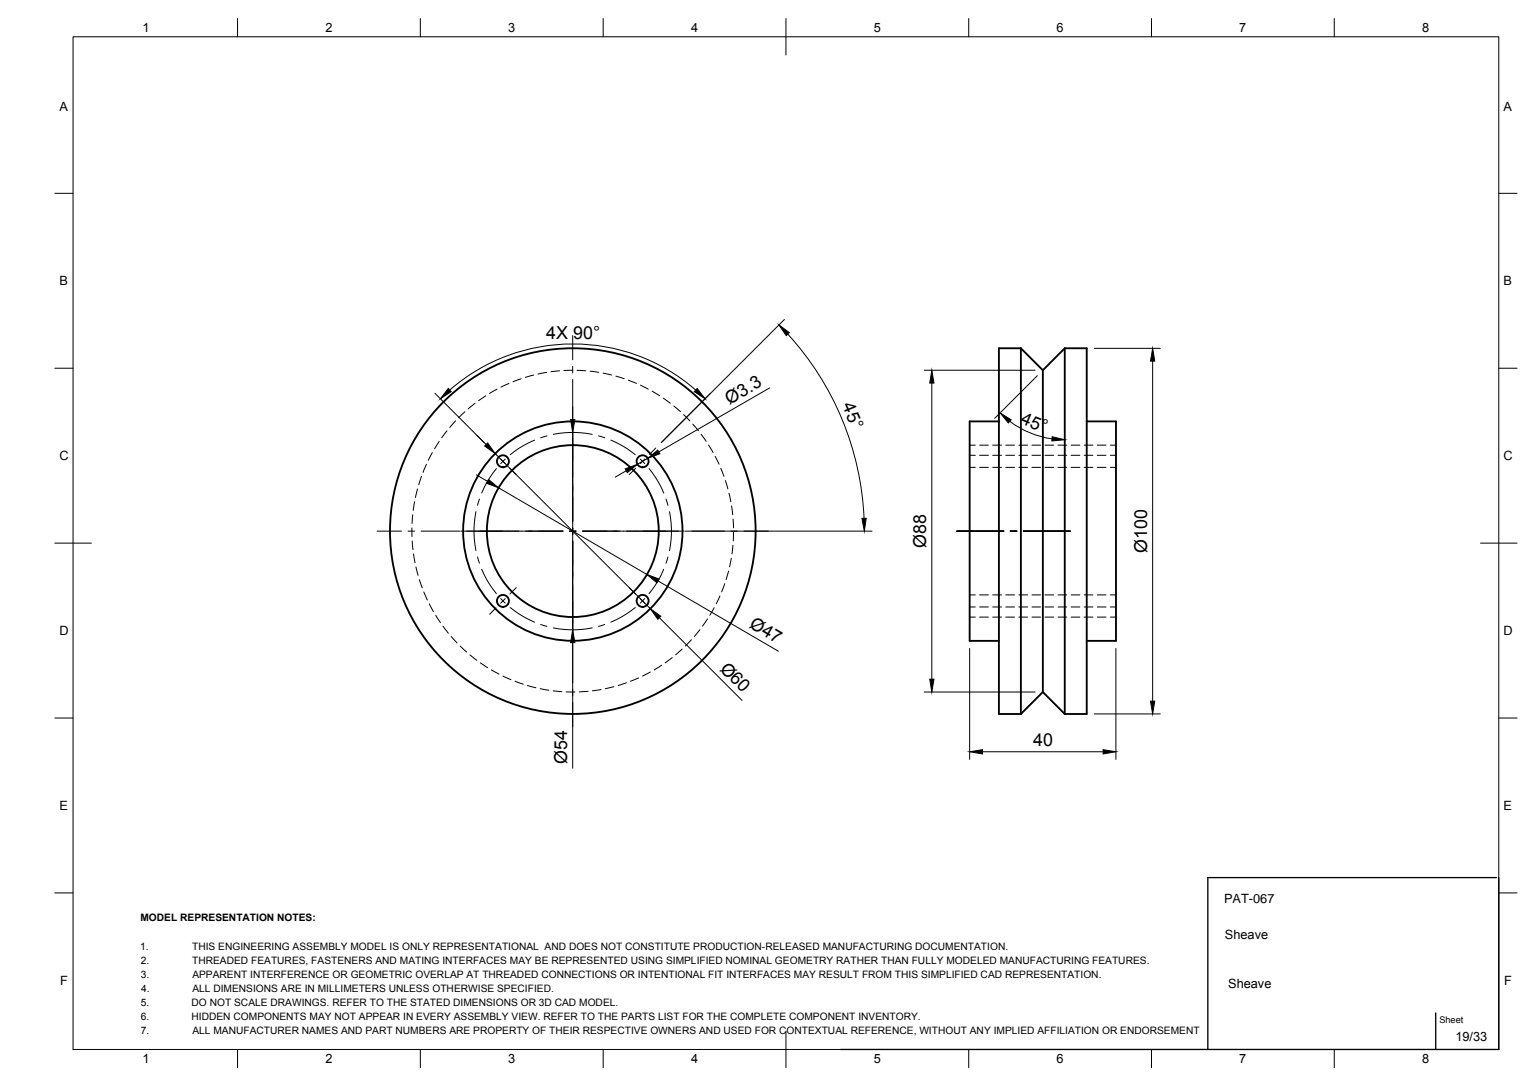
ISO-10303-21;
HEADER;
/* Generated by software containing ST-Developer
 * from STEP Tools, Inc. (www.steptools.com) 
 */

FILE_DESCRIPTION(
/* description */ ('Lifting hook block with sheave'),
/* implementation_level */ '2;1');

FILE_NAME(
/* name */ 'Sheave.step',
/* time_stamp */ '2026-10-28T03:23:54-07:00',
/* author */ (''),
/* organization */ (''),
/* preprocessor_version */ 'ST-DEVELOPER v20.2',
/* originating_system */ 'Autodesk Translation Framework v15.17.0.0',
/* authorisation */ '');

FILE_SCHEMA (('AUTOMOTIVE_DESIGN { 1 0 10303 214 3 1 1 }'));
ENDSEC;

DATA;
#10=MECHANICAL_DESIGN_GEOMETRIC_PRESENTATION_REPRESENTATION('',(#367),#9391);
#276=CONICAL_SURFACE('',#5601,4.7,0.785398163397448);
#277=CONICAL_SURFACE('',#5604,4.7,0.785398163397448);
#307=SHAPE_REPRESENTATION_RELATIONSHIP('SRR','None',#9539,#337);
#337=ADVANCED_BREP_SHAPE_REPRESENTATION('',(#403),#9374);
#367=STYLED_ITEM('',(#9752),#403);
#403=MANIFOLD_SOLID_BREP('Body1',#4905);
#599=LINE('',#8315,#887);
#600=LINE('',#8321,#888);
#601=LINE('',#8327,#889);
#602=LINE('',#8333,#890);
#603=LINE('',#8339,#891);
#604=LINE('',#8344,#892);
#605=LINE('',#8348,#893);
#606=LINE('',#8358,#894);
#607=LINE('',#8361,#895);
#608=LINE('',#8367,#896);
#609=LINE('',#8372,#897);
#887=VECTOR('',#6768,0.165);
#888=VECTOR('',#6775,0.165);
#889=VECTOR('',#6782,0.165);
#890=VECTOR('',#6789,0.165);
#891=VECTOR('',#6796,4.7);
#892=VECTOR('',#6803,4.7);
#893=VECTOR('',#6808,5.);
#894=VECTOR('',#6821,5.);
#895=VECTOR('',#6824,3.);
#896=VECTOR('',#6831,2.35);
#897=VECTOR('',#6838,3.);
#1056=CYLINDRICAL_SURFACE('',#5589,0.165);
#1057=CYLINDRICAL_SURFACE('',#5592,0.165);
#1058=CYLINDRICAL_SURFACE('',#5595,0.165);
#1059=CYLINDRICAL_SURFACE('',#5598,0.165);
#1060=CYLINDRICAL_SURFACE('',#5606,5.);
#1061=CYLINDRICAL_SURFACE('',#5613,5.);
#1062=CYLINDRICAL_SURFACE('',#5614,3.);
#1063=CYLINDRICAL_SURFACE('',#5616,2.35);
#1064=CYLINDRICAL_SURFACE('',#5619,3.);
#1166=FACE_BOUND('',#1726,.T.);
#1167=FACE_BOUND('',#1728,.T.);
#1168=FACE_BOUND('',#1734,.T.);
#1169=FACE_BOUND('',#1735,.T.);
#1170=FACE_BOUND('',#1736,.T.);
#1171=FACE_BOUND('',#1737,.T.);
#1172=FACE_BOUND('',#1738,.T.);
#1173=FACE_BOUND('',#1740,.T.);
#1174=FACE_BOUND('',#1741,.T.);
#1175=FACE_BOUND('',#1742,.T.);
#1176=FACE_BOUND('',#1743,.T.);
#1177=FACE_BOUND('',#1744,.T.);
#1370=FACE_OUTER_BOUND('',#1718,.T.);
#1371=FACE_OUTER_BOUND('',#1719,.T.);
#1372=FACE_OUTER_BOUND('',#1720,.T.);
#1373=FACE_OUTER_BOUND('',#1721,.T.);
#1374=FACE_OUTER_BOUND('',#1722,.T.);
#1375=FACE_OUTER_BOUND('',#1723,.T.);
#1376=FACE_OUTER_BOUND('',#1724,.T.);
#1377=FACE_OUTER_BOUND('',#1725,.T.);
#1378=FACE_OUTER_BOUND('',#1727,.T.);
#1379=FACE_OUTER_BOUND('',#1729,.T.);
#1380=FACE_OUTER_BOUND('',#1730,.T.);
#1381=FACE_OUTER_BOUND('',#1731,.T.);
#1382=FACE_OUTER_BOUND('',#1732,.T.);
#1383=FACE_OUTER_BOUND('',#1733,.T.);
#1384=FACE_OUTER_BOUND('',#1739,.T.);
#1718=EDGE_LOOP('',(#3878,#3879,#3880,#3881));
#1719=EDGE_LOOP('',(#3882,#3883,#3884,#3885));
#1720=EDGE_LOOP('',(#3886,#3887,#3888,#3889));
#1721=EDGE_LOOP('',(#3890,#3891,#3892,#3893));
#1722=EDGE_LOOP('',(#3894,#3895,#3896,#3897));
#1723=EDGE_LOOP('',(#3898,#3899,#3900,#3901));
#1724=EDGE_LOOP('',(#3902,#3903,#3904,#3905));
#1725=EDGE_LOOP('',(#3906));
#1726=EDGE_LOOP('',(#3907));
#1727=EDGE_LOOP('',(#3908));
#1728=EDGE_LOOP('',(#3909));
#1729=EDGE_LOOP('',(#3910,#3911,#3912,#3913));
#1730=EDGE_LOOP('',(#3914,#3915,#3916,#3917));
#1731=EDGE_LOOP('',(#3918,#3919,#3920,#3921));
#1732=EDGE_LOOP('',(#3922,#3923,#3924,#3925));
#1733=EDGE_LOOP('',(#3926));
#1734=EDGE_LOOP('',(#3927));
#1735=EDGE_LOOP('',(#3928));
#1736=EDGE_LOOP('',(#3929));
#1737=EDGE_LOOP('',(#3930));
#1738=EDGE_LOOP('',(#3931));
#1739=EDGE_LOOP('',(#3932));
#1740=EDGE_LOOP('',(#3933));
#1741=EDGE_LOOP('',(#3934));
#1742=EDGE_LOOP('',(#3935));
#1743=EDGE_LOOP('',(#3936));
#1744=EDGE_LOOP('',(#3937));
#2052=CIRCLE('',#5590,0.165);
#2053=CIRCLE('',#5591,0.165);
#2054=CIRCLE('',#5593,0.165);
#2055=CIRCLE('',#5594,0.165);
#2056=CIRCLE('',#5596,0.165);
#2057=CIRCLE('',#5597,0.165);
#2058=CIRCLE('',#5599,0.165);
#2059=CIRCLE('',#5600,0.165);
#2060=CIRCLE('',#5602,4.4);
#2061=CIRCLE('',#5603,5.);
#2062=CIRCLE('',#5605,5.);
#2063=CIRCLE('',#5607,5.);
#2064=CIRCLE('',#5609,3.);
#2065=CIRCLE('',#5611,5.);
#2066=CIRCLE('',#5612,3.);
#2067=CIRCLE('',#5615,3.);
#2068=CIRCLE('',#5617,2.35);
#2069=CIRCLE('',#5618,2.35);
#2070=CIRCLE('',#5620,3.);
#2421=VERTEX_POINT('',#8312);
#2422=VERTEX_POINT('',#8314);
#2423=VERTEX_POINT('',#8318);
#2424=VERTEX_POINT('',#8320);
#2425=VERTEX_POINT('',#8324);
#2426=VERTEX_POINT('',#8326);
#2427=VERTEX_POINT('',#8330);
#2428=VERTEX_POINT('',#8332);
#2429=VERTEX_POINT('',#8336);
#2430=VERTEX_POINT('',#8338);
#2431=VERTEX_POINT('',#8342);
#2432=VERTEX_POINT('',#8346);
#2433=VERTEX_POINT('',#8350);
#2434=VERTEX_POINT('',#8353);
#2435=VERTEX_POINT('',#8355);
#2436=VERTEX_POINT('',#8360);
#2437=VERTEX_POINT('',#8364);
#2438=VERTEX_POINT('',#8366);
#2439=VERTEX_POINT('',#8370);
#2943=EDGE_CURVE('',#2421,#2421,#2052,.T.);
#2944=EDGE_CURVE('',#2421,#2422,#599,.T.);
#2945=EDGE_CURVE('',#2422,#2422,#2053,.T.);
#2946=EDGE_CURVE('',#2423,#2423,#2054,.T.);
#2947=EDGE_CURVE('',#2423,#2424,#600,.T.);
#2948=EDGE_CURVE('',#2424,#2424,#2055,.T.);
#2949=EDGE_CURVE('',#2425,#2425,#2056,.T.);
#2950=EDGE_CURVE('',#2425,#2426,#601,.T.);
#2951=EDGE_CURVE('',#2426,#2426,#2057,.T.);
#2952=EDGE_CURVE('',#2427,#2427,#2058,.T.);
#2953=EDGE_CURVE('',#2427,#2428,#602,.T.);
#2954=EDGE_CURVE('',#2428,#2428,#2059,.T.);
#2955=EDGE_CURVE('',#2429,#2429,#2060,.T.);
#2956=EDGE_CURVE('',#2429,#2430,#603,.T.);
#2957=EDGE_CURVE('',#2430,#2430,#2061,.T.);
#2958=EDGE_CURVE('',#2431,#2431,#2062,.T.);
#2959=EDGE_CURVE('',#2431,#2429,#604,.T.);
#2960=EDGE_CURVE('',#2432,#2432,#2063,.T.);
#2961=EDGE_CURVE('',#2432,#2431,#605,.T.);
#2962=EDGE_CURVE('',#2433,#2433,#2064,.T.);
#2963=EDGE_CURVE('',#2434,#2434,#2065,.T.);
#2964=EDGE_CURVE('',#2435,#2435,#2066,.T.);
#2965=EDGE_CURVE('',#2430,#2434,#606,.T.);
#2966=EDGE_CURVE('',#2435,#2436,#607,.T.);
#2967=EDGE_CURVE('',#2436,#2436,#2067,.T.);
#2968=EDGE_CURVE('',#2437,#2437,#2068,.T.);
#2969=EDGE_CURVE('',#2437,#2438,#608,.T.);
#2970=EDGE_CURVE('',#2438,#2438,#2069,.T.);
#2971=EDGE_CURVE('',#2439,#2439,#2070,.T.);
#2972=EDGE_CURVE('',#2439,#2433,#609,.T.);
#3878=ORIENTED_EDGE('',*,*,#2943,.F.);
#3879=ORIENTED_EDGE('',*,*,#2944,.T.);
#3880=ORIENTED_EDGE('',*,*,#2945,.F.);
#3881=ORIENTED_EDGE('',*,*,#2944,.F.);
#3882=ORIENTED_EDGE('',*,*,#2946,.F.);
#3883=ORIENTED_EDGE('',*,*,#2947,.T.);
#3884=ORIENTED_EDGE('',*,*,#2948,.F.);
#3885=ORIENTED_EDGE('',*,*,#2947,.F.);
#3886=ORIENTED_EDGE('',*,*,#2949,.F.);
#3887=ORIENTED_EDGE('',*,*,#2950,.T.);
#3888=ORIENTED_EDGE('',*,*,#2951,.F.);
#3889=ORIENTED_EDGE('',*,*,#2950,.F.);
#3890=ORIENTED_EDGE('',*,*,#2952,.F.);
#3891=ORIENTED_EDGE('',*,*,#2953,.T.);
#3892=ORIENTED_EDGE('',*,*,#2954,.F.);
#3893=ORIENTED_EDGE('',*,*,#2953,.F.);
#3894=ORIENTED_EDGE('',*,*,#2955,.T.);
#3895=ORIENTED_EDGE('',*,*,#2956,.T.);
#3896=ORIENTED_EDGE('',*,*,#2957,.F.);
#3897=ORIENTED_EDGE('',*,*,#2956,.F.);
#3898=ORIENTED_EDGE('',*,*,#2958,.F.);
#3899=ORIENTED_EDGE('',*,*,#2959,.T.);
#3900=ORIENTED_EDGE('',*,*,#2955,.F.);
#3901=ORIENTED_EDGE('',*,*,#2959,.F.);
#3902=ORIENTED_EDGE('',*,*,#2960,.F.);
#3903=ORIENTED_EDGE('',*,*,#2961,.T.);
#3904=ORIENTED_EDGE('',*,*,#2958,.T.);
#3905=ORIENTED_EDGE('',*,*,#2961,.F.);
#3906=ORIENTED_EDGE('',*,*,#2960,.T.);
#3907=ORIENTED_EDGE('',*,*,#2962,.F.);
#3908=ORIENTED_EDGE('',*,*,#2963,.F.);
#3909=ORIENTED_EDGE('',*,*,#2964,.F.);
#3910=ORIENTED_EDGE('',*,*,#2957,.T.);
#3911=ORIENTED_EDGE('',*,*,#2965,.T.);
#3912=ORIENTED_EDGE('',*,*,#2963,.T.);
#3913=ORIENTED_EDGE('',*,*,#2965,.F.);
#3914=ORIENTED_EDGE('',*,*,#2964,.T.);
#3915=ORIENTED_EDGE('',*,*,#2966,.T.);
#3916=ORIENTED_EDGE('',*,*,#2967,.T.);
#3917=ORIENTED_EDGE('',*,*,#2966,.F.);
#3918=ORIENTED_EDGE('',*,*,#2968,.F.);
#3919=ORIENTED_EDGE('',*,*,#2969,.T.);
#3920=ORIENTED_EDGE('',*,*,#2970,.T.);
#3921=ORIENTED_EDGE('',*,*,#2969,.F.);
#3922=ORIENTED_EDGE('',*,*,#2971,.F.);
#3923=ORIENTED_EDGE('',*,*,#2972,.T.);
#3924=ORIENTED_EDGE('',*,*,#2962,.T.);
#3925=ORIENTED_EDGE('',*,*,#2972,.F.);
#3926=ORIENTED_EDGE('',*,*,#2971,.T.);
#3927=ORIENTED_EDGE('',*,*,#2968,.T.);
#3928=ORIENTED_EDGE('',*,*,#2954,.T.);
#3929=ORIENTED_EDGE('',*,*,#2951,.T.);
#3930=ORIENTED_EDGE('',*,*,#2948,.T.);
#3931=ORIENTED_EDGE('',*,*,#2945,.T.);
#3932=ORIENTED_EDGE('',*,*,#2967,.F.);
#3933=ORIENTED_EDGE('',*,*,#2970,.F.);
#3934=ORIENTED_EDGE('',*,*,#2952,.T.);
#3935=ORIENTED_EDGE('',*,*,#2949,.T.);
#3936=ORIENTED_EDGE('',*,*,#2946,.T.);
#3937=ORIENTED_EDGE('',*,*,#2943,.T.);
#4535=PLANE('',#5608);
#4536=PLANE('',#5610);
#4537=PLANE('',#5621);
#4538=PLANE('',#5622);
#4746=ADVANCED_FACE('',(#1370),#1056,.F.);
#4747=ADVANCED_FACE('',(#1371),#1057,.F.);
#4748=ADVANCED_FACE('',(#1372),#1058,.F.);
#4749=ADVANCED_FACE('',(#1373),#1059,.F.);
#4750=ADVANCED_FACE('',(#1374),#276,.T.);
#4751=ADVANCED_FACE('',(#1375),#277,.T.);
#4752=ADVANCED_FACE('',(#1376),#1060,.T.);
#4753=ADVANCED_FACE('',(#1377,#1166),#4535,.T.);
#4754=ADVANCED_FACE('',(#1378,#1167),#4536,.F.);
#4755=ADVANCED_FACE('',(#1379),#1061,.T.);
#4756=ADVANCED_FACE('',(#1380),#1062,.T.);
#4757=ADVANCED_FACE('',(#1381),#1063,.F.);
#4758=ADVANCED_FACE('',(#1382),#1064,.T.);
#4759=ADVANCED_FACE('',(#1383,#1168,#1169,#1170,#1171,#1172),#4537,.T.);
#4760=ADVANCED_FACE('',(#1384,#1173,#1174,#1175,#1176,#1177),#4538,.F.);
#4905=CLOSED_SHELL('',(#4746,#4747,#4748,#4749,#4750,#4751,#4752,#4753,
#4754,#4755,#4756,#4757,#4758,#4759,#4760));
#5588=AXIS2_PLACEMENT_3D('',#8310,#6762,#6763);
#5589=AXIS2_PLACEMENT_3D('',#8311,#6764,#6765);
#5590=AXIS2_PLACEMENT_3D('',#8313,#6766,#6767);
#5591=AXIS2_PLACEMENT_3D('',#8316,#6769,#6770);
#5592=AXIS2_PLACEMENT_3D('',#8317,#6771,#6772);
#5593=AXIS2_PLACEMENT_3D('',#8319,#6773,#6774);
#5594=AXIS2_PLACEMENT_3D('',#8322,#6776,#6777);
#5595=AXIS2_PLACEMENT_3D('',#8323,#6778,#6779);
#5596=AXIS2_PLACEMENT_3D('',#8325,#6780,#6781);
#5597=AXIS2_PLACEMENT_3D('',#8328,#6783,#6784);
#5598=AXIS2_PLACEMENT_3D('',#8329,#6785,#6786);
#5599=AXIS2_PLACEMENT_3D('',#8331,#6787,#6788);
#5600=AXIS2_PLACEMENT_3D('',#8334,#6790,#6791);
#5601=AXIS2_PLACEMENT_3D('',#8335,#6792,#6793);
#5602=AXIS2_PLACEMENT_3D('',#8337,#6794,#6795);
#5603=AXIS2_PLACEMENT_3D('',#8340,#6797,#6798);
#5604=AXIS2_PLACEMENT_3D('',#8341,#6799,#6800);
#5605=AXIS2_PLACEMENT_3D('',#8343,#6801,#6802);
#5606=AXIS2_PLACEMENT_3D('',#8345,#6804,#6805);
#5607=AXIS2_PLACEMENT_3D('',#8347,#6806,#6807);
#5608=AXIS2_PLACEMENT_3D('',#8349,#6809,#6810);
#5609=AXIS2_PLACEMENT_3D('',#8351,#6811,#6812);
#5610=AXIS2_PLACEMENT_3D('',#8352,#6813,#6814);
#5611=AXIS2_PLACEMENT_3D('',#8354,#6815,#6816);
#5612=AXIS2_PLACEMENT_3D('',#8356,#6817,#6818);
#5613=AXIS2_PLACEMENT_3D('',#8357,#6819,#6820);
#5614=AXIS2_PLACEMENT_3D('',#8359,#6822,#6823);
#5615=AXIS2_PLACEMENT_3D('',#8362,#6825,#6826);
#5616=AXIS2_PLACEMENT_3D('',#8363,#6827,#6828);
#5617=AXIS2_PLACEMENT_3D('',#8365,#6829,#6830);
#5618=AXIS2_PLACEMENT_3D('',#8368,#6832,#6833);
#5619=AXIS2_PLACEMENT_3D('',#8369,#6834,#6835);
#5620=AXIS2_PLACEMENT_3D('',#8371,#6836,#6837);
#5621=AXIS2_PLACEMENT_3D('',#8373,#6839,#6840);
#5622=AXIS2_PLACEMENT_3D('',#8374,#6841,#6842);
#6762=DIRECTION('axis',(0.,0.,1.));
#6763=DIRECTION('refdir',(1.,0.,0.));
#6764=DIRECTION('center_axis',(0.,1.,0.));
#6765=DIRECTION('ref_axis',(1.,0.,0.));
#6766=DIRECTION('center_axis',(0.,1.,0.));
#6767=DIRECTION('ref_axis',(1.,0.,0.));
#6768=DIRECTION('',(0.,1.,0.));
#6769=DIRECTION('center_axis',(0.,-1.,0.));
#6770=DIRECTION('ref_axis',(1.,0.,0.));
#6771=DIRECTION('center_axis',(0.,1.,0.));
#6772=DIRECTION('ref_axis',(1.,0.,0.));
#6773=DIRECTION('center_axis',(0.,1.,0.));
#6774=DIRECTION('ref_axis',(1.,0.,0.));
#6775=DIRECTION('',(0.,1.,0.));
#6776=DIRECTION('center_axis',(0.,-1.,0.));
#6777=DIRECTION('ref_axis',(1.,0.,0.));
#6778=DIRECTION('center_axis',(0.,1.,0.));
#6779=DIRECTION('ref_axis',(1.,0.,0.));
#6780=DIRECTION('center_axis',(0.,1.,0.));
#6781=DIRECTION('ref_axis',(1.,0.,0.));
#6782=DIRECTION('',(0.,1.,0.));
#6783=DIRECTION('center_axis',(0.,-1.,0.));
#6784=DIRECTION('ref_axis',(1.,0.,0.));
#6785=DIRECTION('center_axis',(0.,1.,0.));
#6786=DIRECTION('ref_axis',(1.,0.,0.));
#6787=DIRECTION('center_axis',(0.,1.,0.));
#6788=DIRECTION('ref_axis',(1.,0.,0.));
#6789=DIRECTION('',(0.,1.,0.));
#6790=DIRECTION('center_axis',(0.,-1.,0.));
#6791=DIRECTION('ref_axis',(1.,0.,0.));
#6792=DIRECTION('center_axis',(0.,-1.,0.));
#6793=DIRECTION('ref_axis',(1.,0.,0.));
#6794=DIRECTION('center_axis',(0.,-1.,0.));
#6795=DIRECTION('ref_axis',(1.,0.,0.));
#6796=DIRECTION('',(-0.707106781186547,-0.707106781186548,-8.65956056235493E-17));
#6797=DIRECTION('center_axis',(0.,-1.,0.));
#6798=DIRECTION('ref_axis',(1.,0.,0.));
#6799=DIRECTION('center_axis',(0.,1.,0.));
#6800=DIRECTION('ref_axis',(1.,0.,0.));
#6801=DIRECTION('center_axis',(0.,1.,0.));
#6802=DIRECTION('ref_axis',(1.,0.,0.));
#6803=DIRECTION('',(0.707106781186547,-0.707106781186548,8.65956056235493E-17));
#6804=DIRECTION('center_axis',(0.,1.,0.));
#6805=DIRECTION('ref_axis',(1.,0.,0.));
#6806=DIRECTION('center_axis',(0.,1.,0.));
#6807=DIRECTION('ref_axis',(1.,0.,0.));
#6808=DIRECTION('',(0.,-1.,0.));
#6809=DIRECTION('center_axis',(0.,1.,0.));
#6810=DIRECTION('ref_axis',(1.,0.,0.));
#6811=DIRECTION('center_axis',(0.,1.,0.));
#6812=DIRECTION('ref_axis',(1.,0.,0.));
#6813=DIRECTION('center_axis',(0.,1.,0.));
#6814=DIRECTION('ref_axis',(1.,0.,0.));
#6815=DIRECTION('center_axis',(0.,1.,0.));
#6816=DIRECTION('ref_axis',(1.,0.,0.));
#6817=DIRECTION('center_axis',(0.,-1.,0.));
#6818=DIRECTION('ref_axis',(1.,0.,0.));
#6819=DIRECTION('center_axis',(0.,1.,0.));
#6820=DIRECTION('ref_axis',(1.,0.,0.));
#6821=DIRECTION('',(0.,-1.,0.));
#6822=DIRECTION('center_axis',(0.,1.,0.));
#6823=DIRECTION('ref_axis',(1.,0.,0.));
#6824=DIRECTION('',(0.,-1.,0.));
#6825=DIRECTION('center_axis',(0.,1.,0.));
#6826=DIRECTION('ref_axis',(1.,0.,0.));
#6827=DIRECTION('center_axis',(0.,1.,0.));
#6828=DIRECTION('ref_axis',(1.,0.,0.));
#6829=DIRECTION('center_axis',(0.,-1.,0.));
#6830=DIRECTION('ref_axis',(1.,0.,0.));
#6831=DIRECTION('',(0.,-1.,0.));
#6832=DIRECTION('center_axis',(0.,-1.,0.));
#6833=DIRECTION('ref_axis',(1.,0.,0.));
#6834=DIRECTION('center_axis',(0.,1.,0.));
#6835=DIRECTION('ref_axis',(1.,0.,0.));
#6836=DIRECTION('center_axis',(0.,1.,0.));
#6837=DIRECTION('ref_axis',(1.,0.,0.));
#6838=DIRECTION('',(0.,-1.,0.));
#6839=DIRECTION('center_axis',(0.,1.,0.));
#6840=DIRECTION('ref_axis',(1.,0.,0.));
#6841=DIRECTION('center_axis',(0.,1.,0.));
#6842=DIRECTION('ref_axis',(1.,0.,0.));
#8310=CARTESIAN_POINT('',(0.,0.,0.));
#8311=CARTESIAN_POINT('Origin',(-1.90918830920368,-2.1,10.0908116907963));
#8312=CARTESIAN_POINT('',(-2.07418830920368,-2.,10.0908116907963));
#8313=CARTESIAN_POINT('Origin',(-1.90918830920368,-2.,10.0908116907963));
#8314=CARTESIAN_POINT('',(-2.07418830920368,2.,10.0908116907963));
#8315=CARTESIAN_POINT('',(-2.07418830920368,-2.1,10.0908116907963));
#8316=CARTESIAN_POINT('Origin',(-1.90918830920368,2.,10.0908116907963));
#8317=CARTESIAN_POINT('Origin',(-1.90918830920368,-2.1,13.9091883092037));
#8318=CARTESIAN_POINT('',(-2.07418830920368,-2.,13.9091883092037));
#8319=CARTESIAN_POINT('Origin',(-1.90918830920368,-2.,13.9091883092037));
#8320=CARTESIAN_POINT('',(-2.07418830920368,2.,13.9091883092037));
#8321=CARTESIAN_POINT('',(-2.07418830920368,-2.1,13.9091883092037));
#8322=CARTESIAN_POINT('Origin',(-1.90918830920368,2.,13.9091883092037));
#8323=CARTESIAN_POINT('Origin',(1.90918830920368,-2.1,13.9091883092037));
#8324=CARTESIAN_POINT('',(1.74418830920368,-2.,13.9091883092037));
#8325=CARTESIAN_POINT('Origin',(1.90918830920368,-2.,13.9091883092037));
#8326=CARTESIAN_POINT('',(1.74418830920368,2.,13.9091883092037));
#8327=CARTESIAN_POINT('',(1.74418830920368,-2.1,13.9091883092037));
#8328=CARTESIAN_POINT('Origin',(1.90918830920368,2.,13.9091883092037));
#8329=CARTESIAN_POINT('Origin',(1.90918830920368,-2.1,10.0908116907963));
#8330=CARTESIAN_POINT('',(1.74418830920368,-2.,10.0908116907963));
#8331=CARTESIAN_POINT('Origin',(1.90918830920368,-2.,10.0908116907963));
#8332=CARTESIAN_POINT('',(1.74418830920368,2.,10.0908116907963));
#8333=CARTESIAN_POINT('',(1.74418830920368,-2.1,10.0908116907963));
#8334=CARTESIAN_POINT('Origin',(1.90918830920368,2.,10.0908116907963));
#8335=CARTESIAN_POINT('Origin',(0.,-0.3,12.));
#8336=CARTESIAN_POINT('',(-4.4,4.44089209850063E-16,12.));
#8337=CARTESIAN_POINT('Origin',(0.,0.,12.));
#8338=CARTESIAN_POINT('',(-5.,-0.6,12.));
#8339=CARTESIAN_POINT('',(-4.7,-0.3,12.));
#8340=CARTESIAN_POINT('Origin',(0.,-0.6,12.));
#8341=CARTESIAN_POINT('Origin',(0.,0.3,12.));
#8342=CARTESIAN_POINT('',(-5.,0.6,12.));
#8343=CARTESIAN_POINT('Origin',(0.,0.6,12.));
#8344=CARTESIAN_POINT('',(-4.7,0.3,12.));
#8345=CARTESIAN_POINT('Origin',(0.,-1.2,12.));
#8346=CARTESIAN_POINT('',(-5.,1.2,12.));
#8347=CARTESIAN_POINT('Origin',(0.,1.2,12.));
#8348=CARTESIAN_POINT('',(-5.,-1.2,12.));
#8349=CARTESIAN_POINT('Origin',(0.,1.2,12.));
#8350=CARTESIAN_POINT('',(-3.,1.2,12.));
#8351=CARTESIAN_POINT('Origin',(0.,1.2,12.));
#8352=CARTESIAN_POINT('Origin',(0.,-1.2,12.));
#8353=CARTESIAN_POINT('',(-5.,-1.2,12.));
#8354=CARTESIAN_POINT('Origin',(0.,-1.2,12.));
#8355=CARTESIAN_POINT('',(-3.,-1.2,12.));
#8356=CARTESIAN_POINT('Origin',(0.,-1.2,12.));
#8357=CARTESIAN_POINT('Origin',(0.,-1.2,12.));
#8358=CARTESIAN_POINT('',(-5.,-1.2,12.));
#8359=CARTESIAN_POINT('Origin',(0.,-2.,12.));
#8360=CARTESIAN_POINT('',(-3.,-2.,12.));
#8361=CARTESIAN_POINT('',(-3.,-2.,12.));
#8362=CARTESIAN_POINT('Origin',(0.,-2.,12.));
#8363=CARTESIAN_POINT('Origin',(0.,-2.,12.));
#8364=CARTESIAN_POINT('',(-2.35,2.,12.));
#8365=CARTESIAN_POINT('Origin',(0.,2.,12.));
#8366=CARTESIAN_POINT('',(-2.35,-2.,12.));
#8367=CARTESIAN_POINT('',(-2.35,-2.,12.));
#8368=CARTESIAN_POINT('Origin',(0.,-2.,12.));
#8369=CARTESIAN_POINT('Origin',(0.,-2.,12.));
#8370=CARTESIAN_POINT('',(-3.,2.,12.));
#8371=CARTESIAN_POINT('Origin',(0.,2.,12.));
#8372=CARTESIAN_POINT('',(-3.,-2.,12.));
#8373=CARTESIAN_POINT('Origin',(0.,2.,12.));
#8374=CARTESIAN_POINT('Origin',(0.,-2.,12.));
#9337=UNCERTAINTY_MEASURE_WITH_UNIT(LENGTH_MEASURE(0.001),#9392,
'DISTANCE_ACCURACY_VALUE',
'Maximum model space distance between geometric entities at asserted c
onnectivities');
#9354=UNCERTAINTY_MEASURE_WITH_UNIT(LENGTH_MEASURE(0.001),#9392,
'DISTANCE_ACCURACY_VALUE',
'Maximum model space distance between geometric entities at asserted c
onnectivities');
#9374=(
GEOMETRIC_REPRESENTATION_CONTEXT(3)
GLOBAL_UNCERTAINTY_ASSIGNED_CONTEXT((#9337))
GLOBAL_UNIT_ASSIGNED_CONTEXT((#9392,#9394,#9395))
REPRESENTATION_CONTEXT('','3D')
);
#9391=(
GEOMETRIC_REPRESENTATION_CONTEXT(3)
GLOBAL_UNCERTAINTY_ASSIGNED_CONTEXT((#9354))
GLOBAL_UNIT_ASSIGNED_CONTEXT((#9392,#9394,#9395))
REPRESENTATION_CONTEXT('','3D')
);
#9392=(
LENGTH_UNIT()
NAMED_UNIT(*)
SI_UNIT(.CENTI.,.METRE.)
);
#9394=(
NAMED_UNIT(*)
PLANE_ANGLE_UNIT()
SI_UNIT($,.RADIAN.)
);
#9395=(
NAMED_UNIT(*)
SI_UNIT($,.STERADIAN.)
SOLID_ANGLE_UNIT()
);
#9415=SHAPE_DEFINITION_REPRESENTATION(#9476,#9539);
#9476=PRODUCT_DEFINITION_SHAPE('',$,#9576);
#9539=SHAPE_REPRESENTATION('',(#5588),#9374);
#9556=PRODUCT_DEFINITION_CONTEXT('part definition',#9666,'design');
#9576=PRODUCT_DEFINITION('Sheave','Sheave',#9612,#9556);
#9612=PRODUCT_DEFINITION_FORMATION('',$,#9687);
#9666=APPLICATION_CONTEXT(
'Core Data for Automotive Mechanical Design Process');
#9667=PRODUCT_CONTEXT('part definition',#9666,'mechanical');
#9687=PRODUCT('Sheave','Sheave','Sheave',(#9667));
#9746=COLOUR_RGB('Sky Blue',0.24,0.69,0.87);
#9747=FILL_AREA_STYLE_COLOUR('',#9746);
#9748=FILL_AREA_STYLE('',(#9747));
#9749=SURFACE_STYLE_FILL_AREA(#9748);
#9750=SURFACE_SIDE_STYLE('',(#9749));
#9751=SURFACE_STYLE_USAGE(.BOTH.,#9750);
#9752=PRESENTATION_STYLE_ASSIGNMENT((#9751));
ENDSEC;
END-ISO-10303-21;
